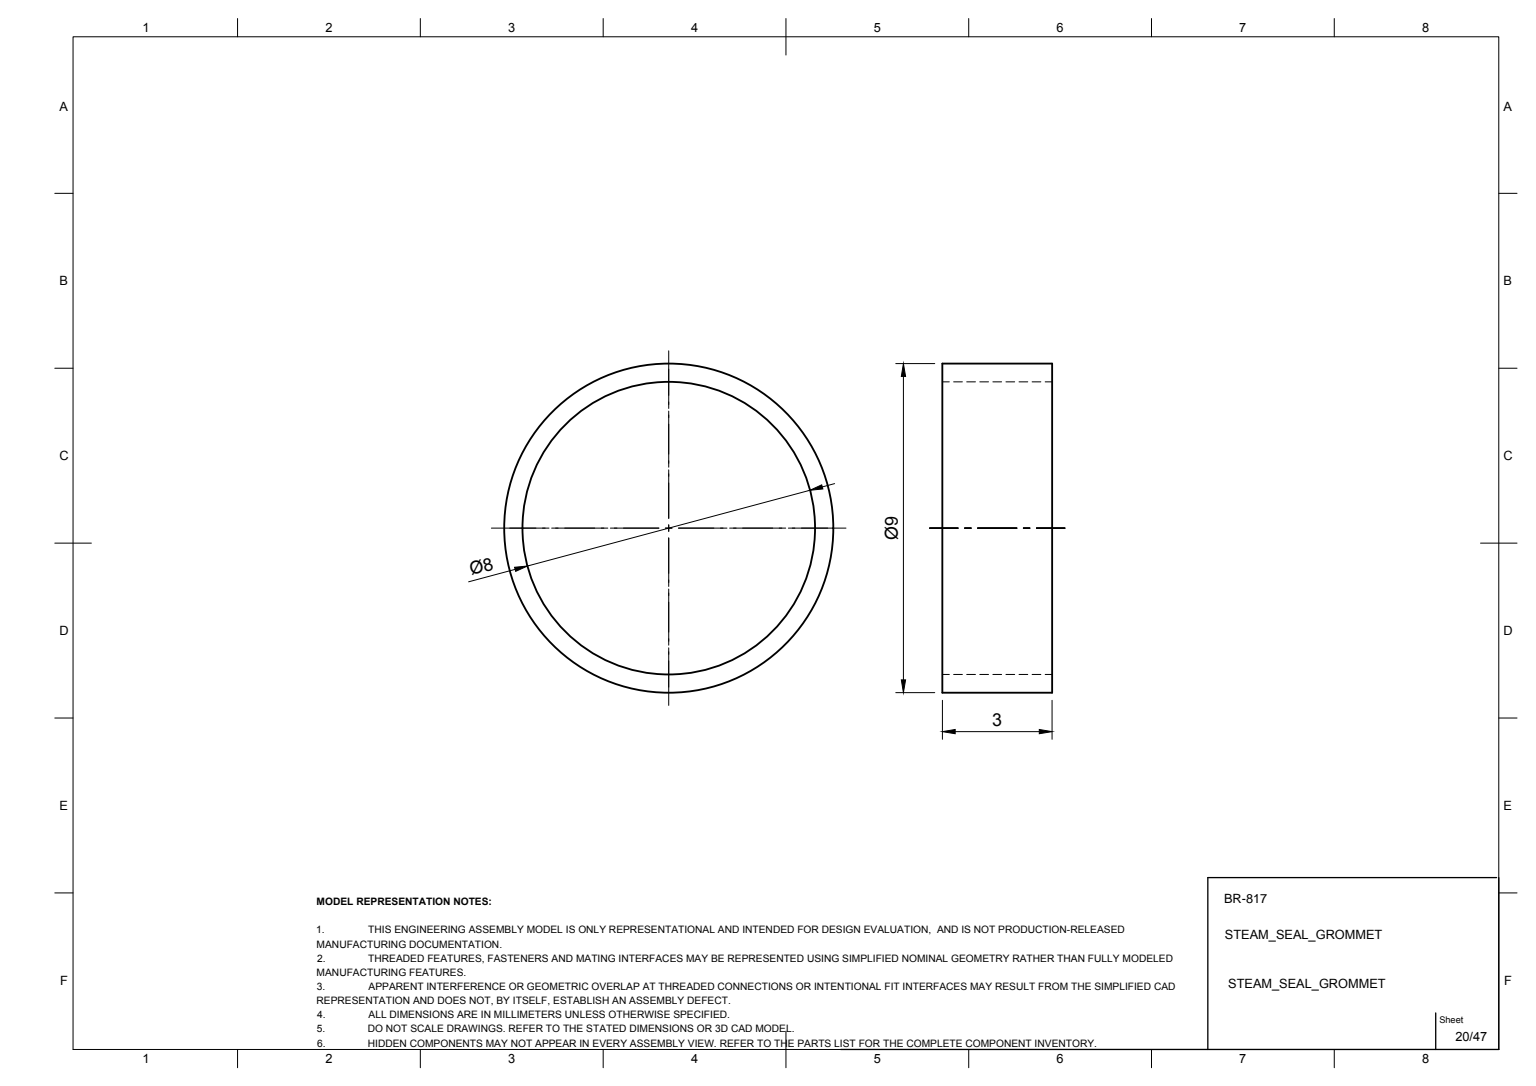
ISO-10303-21;
HEADER;
FILE_DESCRIPTION((''),'2;1');
FILE_NAME('STEAM_SEAL_GROMMET.step','2026-10-01T22:07:29-07:00',(''),(''),'','','');
FILE_SCHEMA (('AUTOMOTIVE_DESIGN { 1 0 10303 214 3 1 1 }'));
ENDSEC;
DATA;
#10=MECHANICAL_DESIGN_GEOMETRIC_PRESENTATION_REPRESENTATION('',(#554),#15484);
#484=SHAPE_REPRESENTATION_RELATIONSHIP('SRR','None',#15633,#519) ;
#519=ADVANCED_BREP_SHAPE_REPRESENTATION('',(#595),#15457) ;
#554=STYLED_ITEM('',(#15837),#595) ;
#595=MANIFOLD_SOLID_BREP('STEAM_SEAL_GROMMET',#8265) ;
#675=CYLINDRICAL_SURFACE('',#8968,0.4) ;
#676=CYLINDRICAL_SURFACE('',#8971,0.45) ;
#861=FACE_BOUND('',#2073,.T.) ;
#862=FACE_BOUND('',#2075,.T.) ;
#993=CIRCLE('',#8969,0.4) ;
#994=CIRCLE('',#8970,0.4) ;
#995=CIRCLE('',#8972,0.45) ;
#996=CIRCLE('',#8973,0.45) ;
#1519=FACE_OUTER_BOUND('',#2070,.T.) ;
#1520=FACE_OUTER_BOUND('',#2071,.T.) ;
#1521=FACE_OUTER_BOUND('',#2072,.T.) ;
#1522=FACE_OUTER_BOUND('',#2074,.T.) ;
#2070=EDGE_LOOP('',(#5901,#5902,#5903,#5904)) ;
#2071=EDGE_LOOP('',(#5905,#5906,#5907,#5908)) ;
#2072=EDGE_LOOP('',(#5909)) ;
#2073=EDGE_LOOP('',(#5910)) ;
#2074=EDGE_LOOP('',(#5911)) ;
#2075=EDGE_LOOP('',(#5912)) ;
#2642=LINE('',#13632,#3116) ;
#2643=LINE('',#13638,#3117) ;
#3116=VECTOR('',#10703,0.4) ;
#3117=VECTOR('',#10710,0.45) ;
#3599=VERTEX_POINT('',#13629) ;
#3600=VERTEX_POINT('',#13631) ;
#3601=VERTEX_POINT('',#13635) ;
#3602=VERTEX_POINT('',#13637) ;
#4455=EDGE_CURVE('',#3599,#3599,#993,.T.) ;
#4456=EDGE_CURVE('',#3599,#3600,#2642,.T.) ;
#4457=EDGE_CURVE('',#3600,#3600,#994,.T.) ;
#4458=EDGE_CURVE('',#3601,#3601,#995,.T.) ;
#4459=EDGE_CURVE('',#3601,#3602,#2643,.T.) ;
#4460=EDGE_CURVE('',#3602,#3602,#996,.T.) ;
#5901=ORIENTED_EDGE('',*,*,#4455,.F.) ;
#5902=ORIENTED_EDGE('',*,*,#4456,.T.) ;
#5903=ORIENTED_EDGE('',*,*,#4457,.F.) ;
#5904=ORIENTED_EDGE('',*,*,#4456,.F.) ;
#5905=ORIENTED_EDGE('',*,*,#4458,.F.) ;
#5906=ORIENTED_EDGE('',*,*,#4459,.T.) ;
#5907=ORIENTED_EDGE('',*,*,#4460,.F.) ;
#5908=ORIENTED_EDGE('',*,*,#4459,.F.) ;
#5909=ORIENTED_EDGE('',*,*,#4460,.T.) ;
#5910=ORIENTED_EDGE('',*,*,#4455,.T.) ;
#5911=ORIENTED_EDGE('',*,*,#4458,.T.) ;
#5912=ORIENTED_EDGE('',*,*,#4457,.T.) ;
#7636=PLANE('',#8974) ;
#7637=PLANE('',#8975) ;
#7906=ADVANCED_FACE('',(#1519),#675,.F.) ;
#7907=ADVANCED_FACE('',(#1520),#676,.T.) ;
#7908=ADVANCED_FACE('',(#1521,#861),#7636,.T.) ;
#7909=ADVANCED_FACE('',(#1522,#862),#7637,.T.) ;
#8265=CLOSED_SHELL('',(#7906,#7907,#7908,#7909)) ;
#8967=AXIS2_PLACEMENT_3D('',#13627,#10697,#10698) ;
#8968=AXIS2_PLACEMENT_3D('',#13628,#10699,#10700) ;
#8969=AXIS2_PLACEMENT_3D('',#13630,#10701,#10702) ;
#8970=AXIS2_PLACEMENT_3D('',#13633,#10704,#10705) ;
#8971=AXIS2_PLACEMENT_3D('',#13634,#10706,#10707) ;
#8972=AXIS2_PLACEMENT_3D('',#13636,#10708,#10709) ;
#8973=AXIS2_PLACEMENT_3D('',#13639,#10711,#10712) ;
#8974=AXIS2_PLACEMENT_3D('',#13640,#10713,#10714) ;
#8975=AXIS2_PLACEMENT_3D('',#13641,#10715,#10716) ;
#10697=DIRECTION('axis',(0.,0.,1.)) ;
#10698=DIRECTION('refdir',(1.,0.,0.)) ;
#10699=DIRECTION('center_axis',(0.,0.,1.)) ;
#10700=DIRECTION('ref_axis',(1.,0.,0.)) ;
#10701=DIRECTION('center_axis',(0.,0.,1.)) ;
#10702=DIRECTION('ref_axis',(1.,0.,0.)) ;
#10703=DIRECTION('',(0.,0.,1.)) ;
#10704=DIRECTION('center_axis',(0.,0.,-1.)) ;
#10705=DIRECTION('ref_axis',(1.,0.,0.)) ;
#10706=DIRECTION('center_axis',(0.,0.,1.)) ;
#10707=DIRECTION('ref_axis',(1.,0.,0.)) ;
#10708=DIRECTION('center_axis',(0.,0.,1.)) ;
#10709=DIRECTION('ref_axis',(1.,0.,0.)) ;
#10710=DIRECTION('',(0.,0.,-1.)) ;
#10711=DIRECTION('center_axis',(0.,0.,-1.)) ;
#10712=DIRECTION('ref_axis',(1.,0.,0.)) ;
#10713=DIRECTION('center_axis',(0.,0.,-1.)) ;
#10714=DIRECTION('ref_axis',(-1.,0.,0.)) ;
#10715=DIRECTION('center_axis',(0.,0.,1.)) ;
#10716=DIRECTION('ref_axis',(1.,0.,0.)) ;
#13627=CARTESIAN_POINT('',(0.,0.,0.)) ;
#13628=CARTESIAN_POINT('Origin',(2.5,1.4,2.15)) ;
#13629=CARTESIAN_POINT('',(2.1,1.4,2.)) ;
#13630=CARTESIAN_POINT('Origin',(2.5,1.4,2.)) ;
#13631=CARTESIAN_POINT('',(2.1,1.4,2.3)) ;
#13632=CARTESIAN_POINT('',(2.1,1.4,2.15)) ;
#13633=CARTESIAN_POINT('Origin',(2.5,1.4,2.3)) ;
#13634=CARTESIAN_POINT('Origin',(2.5,1.4,2.15)) ;
#13635=CARTESIAN_POINT('',(2.05,1.4,2.3)) ;
#13636=CARTESIAN_POINT('Origin',(2.5,1.4,2.3)) ;
#13637=CARTESIAN_POINT('',(2.05,1.4,2.)) ;
#13638=CARTESIAN_POINT('',(2.05,1.4,2.15)) ;
#13639=CARTESIAN_POINT('Origin',(2.5,1.4,2.)) ;
#13640=CARTESIAN_POINT('Origin',(2.5,1.4,2.)) ;
#13641=CARTESIAN_POINT('Origin',(2.5,1.4,2.3)) ;
#15414=UNCERTAINTY_MEASURE_WITH_UNIT(LENGTH_MEASURE(0.001),#15485,
'DISTANCE_ACCURACY_VALUE',
'Maximum model space distance between geometric entities at asserted c
onnectivities') ;
#15441=UNCERTAINTY_MEASURE_WITH_UNIT(LENGTH_MEASURE(0.001),#15485,
'DISTANCE_ACCURACY_VALUE',
'Maximum model space distance between geometric entities at asserted c
onnectivities') ;
#15457=(
GEOMETRIC_REPRESENTATION_CONTEXT(3)
GLOBAL_UNCERTAINTY_ASSIGNED_CONTEXT((#15414))
GLOBAL_UNIT_ASSIGNED_CONTEXT((#15485,#15487,#15488))
REPRESENTATION_CONTEXT('','3D')
) ;
#15484=(
GEOMETRIC_REPRESENTATION_CONTEXT(3)
GLOBAL_UNCERTAINTY_ASSIGNED_CONTEXT((#15441))
GLOBAL_UNIT_ASSIGNED_CONTEXT((#15485,#15487,#15488))
REPRESENTATION_CONTEXT('','3D')
) ;
#15485=(
LENGTH_UNIT()
NAMED_UNIT(*)
SI_UNIT(.CENTI.,.METRE.)
) ;
#15487=(
NAMED_UNIT(*)
PLANE_ANGLE_UNIT()
SI_UNIT($,.RADIAN.)
) ;
#15488=(
NAMED_UNIT(*)
SI_UNIT($,.STERADIAN.)
SOLID_ANGLE_UNIT()
) ;
#15504=SHAPE_DEFINITION_REPRESENTATION(#15552,#15633) ;
#15552=PRODUCT_DEFINITION_SHAPE('',$,#15676) ;
#15633=SHAPE_REPRESENTATION('',(#8967),#15457) ;
#15660=PRODUCT_DEFINITION_CONTEXT('part definition',#15788,'design') ;
#15676=PRODUCT_DEFINITION('STEAM_SEAL_GROMMET',
'STEAM_SEAL_GROMMET',#15718,#15660) ;
#15718=PRODUCT_DEFINITION_FORMATION('',$,#15805) ;
#15788=APPLICATION_CONTEXT(
'Core Data for Automotive Mechanical Design Process') ;
#15789=PRODUCT_CONTEXT('part definition',#15788,'mechanical') ;
#15805=PRODUCT('STEAM_SEAL_GROMMET','STEAM_SEAL_GROMMET',$,(#15789)) ;
#15837=PRESENTATION_STYLE_ASSIGNMENT((#15849)) ;
#15849=SURFACE_STYLE_USAGE(.BOTH.,#15861) ;
#15861=SURFACE_SIDE_STYLE('',(#15873)) ;
#15873=SURFACE_STYLE_FILL_AREA(#15885) ;
#15885=FILL_AREA_STYLE('Silicone (White)',(#15897)) ;
#15897=FILL_AREA_STYLE_COLOUR('Silicone (White)',#15909) ;
#15909=COLOUR_RGB('Silicone (White)', 0.09019608, 0.27058824, 0.51372549) ;
ENDSEC;
END-ISO-10303-21;
